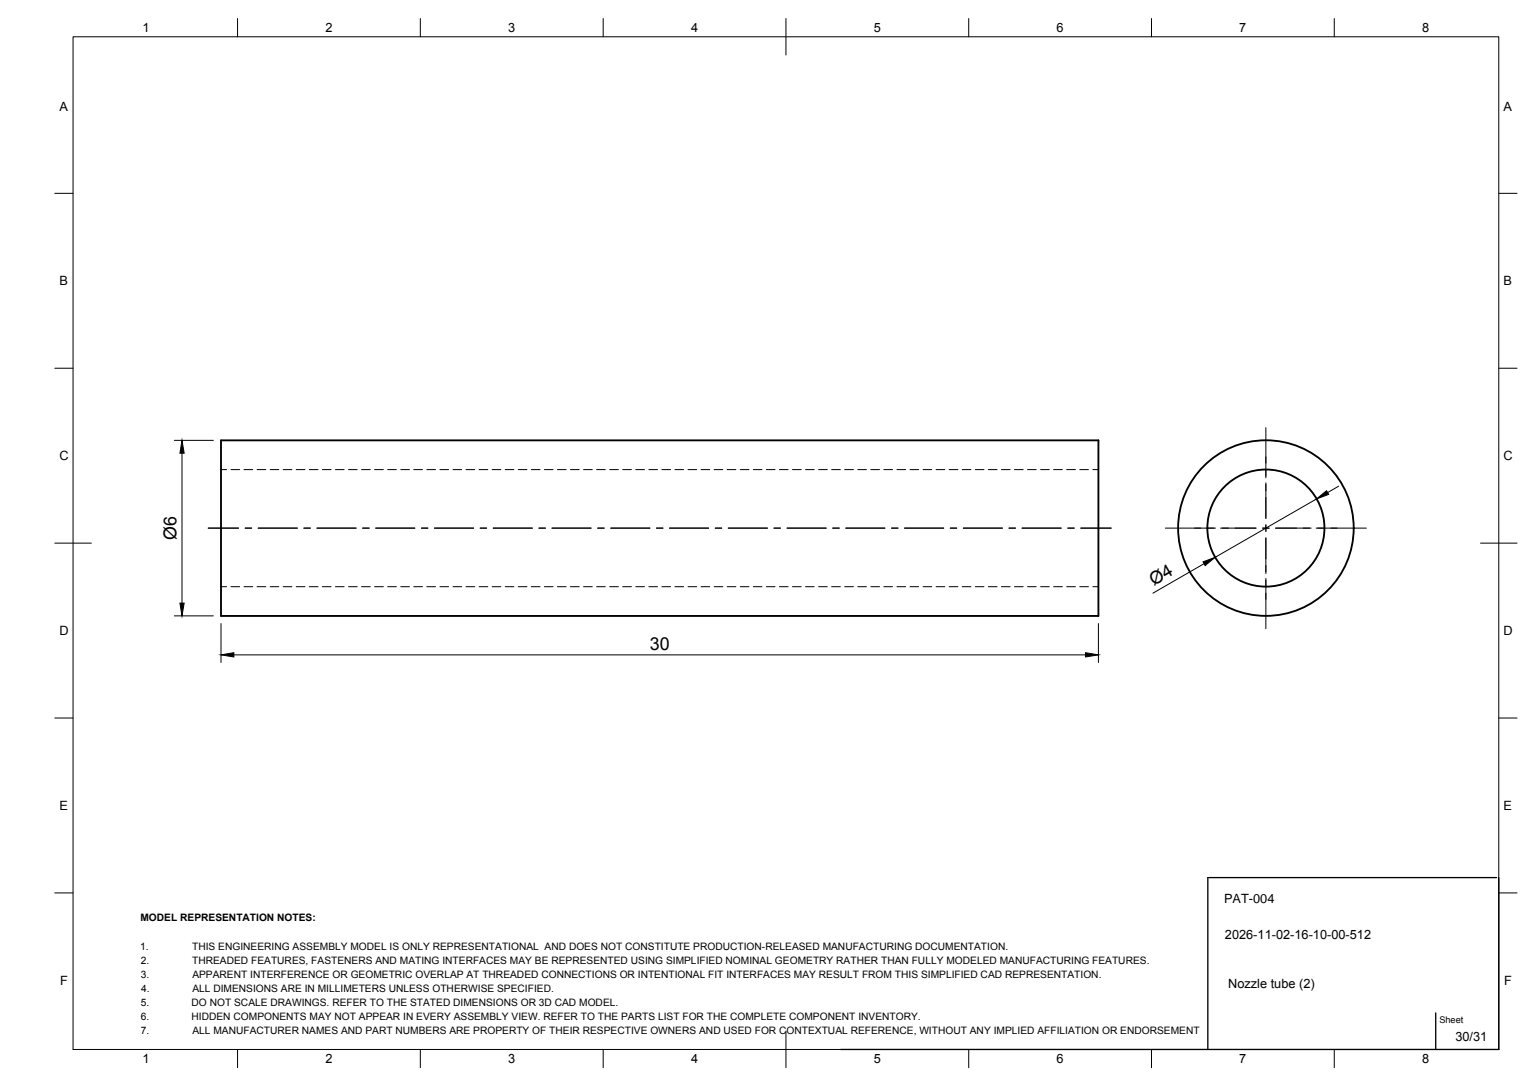
ISO-10303-21;
HEADER;
/* Generated by software containing ST-Developer
 * from STEP Tools, Inc. (www.steptools.com) 
 */

FILE_DESCRIPTION(
/* description */ ('Air blow-off nozzle station'),
/* implementation_level */ '2;1');

FILE_NAME(
/* name */ 'Nozzle tube (2).step',
/* time_stamp */ '2026-10-27T10:53:54-07:00',
/* author */ (''),
/* organization */ (''),
/* preprocessor_version */ 'ST-DEVELOPER v20.2',
/* originating_system */ 'Autodesk Translation Framework v15.17.0.0',
/* authorisation */ '');

FILE_SCHEMA (('AUTOMOTIVE_DESIGN { 1 0 10303 214 3 1 1 }'));
ENDSEC;

DATA;
#10=MECHANICAL_DESIGN_GEOMETRIC_PRESENTATION_REPRESENTATION('',(#258),#7897);
#208=SHAPE_REPRESENTATION_RELATIONSHIP('SRR','None',#8025,#233);
#233=ADVANCED_BREP_SHAPE_REPRESENTATION('',(#281),#7892);
#258=STYLED_ITEM('',(#8206),#281);
#281=MANIFOLD_SOLID_BREP('Body1',#4309);
#357=FACE_BOUND('',#1094,.T.);
#358=FACE_BOUND('',#1096,.T.);
#520=PLANE('',#4997);
#521=PLANE('',#4998);
#763=FACE_OUTER_BOUND('',#1091,.T.);
#764=FACE_OUTER_BOUND('',#1092,.T.);
#765=FACE_OUTER_BOUND('',#1093,.T.);
#766=FACE_OUTER_BOUND('',#1095,.T.);
#1091=EDGE_LOOP('',(#3845,#3846,#3847,#3848));
#1092=EDGE_LOOP('',(#3849,#3850,#3851,#3852));
#1093=EDGE_LOOP('',(#3853));
#1094=EDGE_LOOP('',(#3854));
#1095=EDGE_LOOP('',(#3855));
#1096=EDGE_LOOP('',(#3856));
#1461=LINE('',#7688,#1815);
#1462=LINE('',#7694,#1816);
#1815=VECTOR('',#6203,0.2);
#1816=VECTOR('',#6210,0.3);
#1981=CIRCLE('',#4992,0.2);
#1982=CIRCLE('',#4993,0.2);
#1983=CIRCLE('',#4995,0.3);
#1984=CIRCLE('',#4996,0.3);
#2328=VERTEX_POINT('',#7685);
#2329=VERTEX_POINT('',#7687);
#2330=VERTEX_POINT('',#7691);
#2331=VERTEX_POINT('',#7693);
#2840=EDGE_CURVE('',#2328,#2328,#1981,.T.);
#2841=EDGE_CURVE('',#2328,#2329,#1461,.T.);
#2842=EDGE_CURVE('',#2329,#2329,#1982,.T.);
#2843=EDGE_CURVE('',#2330,#2330,#1983,.T.);
#2844=EDGE_CURVE('',#2330,#2331,#1462,.T.);
#2845=EDGE_CURVE('',#2331,#2331,#1984,.T.);
#3845=ORIENTED_EDGE('',*,*,#2840,.F.);
#3846=ORIENTED_EDGE('',*,*,#2841,.T.);
#3847=ORIENTED_EDGE('',*,*,#2842,.T.);
#3848=ORIENTED_EDGE('',*,*,#2841,.F.);
#3849=ORIENTED_EDGE('',*,*,#2843,.F.);
#3850=ORIENTED_EDGE('',*,*,#2844,.T.);
#3851=ORIENTED_EDGE('',*,*,#2845,.T.);
#3852=ORIENTED_EDGE('',*,*,#2844,.F.);
#3853=ORIENTED_EDGE('',*,*,#2843,.T.);
#3854=ORIENTED_EDGE('',*,*,#2840,.T.);
#3855=ORIENTED_EDGE('',*,*,#2845,.F.);
#3856=ORIENTED_EDGE('',*,*,#2842,.F.);
#4017=CYLINDRICAL_SURFACE('',#4991,0.2);
#4018=CYLINDRICAL_SURFACE('',#4994,0.3);
#4253=ADVANCED_FACE('',(#763),#4017,.F.);
#4254=ADVANCED_FACE('',(#764),#4018,.T.);
#4255=ADVANCED_FACE('',(#765,#357),#520,.T.);
#4256=ADVANCED_FACE('',(#766,#358),#521,.F.);
#4309=CLOSED_SHELL('',(#4253,#4254,#4255,#4256));
#4990=AXIS2_PLACEMENT_3D('',#7683,#6197,#6198);
#4991=AXIS2_PLACEMENT_3D('',#7684,#6199,#6200);
#4992=AXIS2_PLACEMENT_3D('',#7686,#6201,#6202);
#4993=AXIS2_PLACEMENT_3D('',#7689,#6204,#6205);
#4994=AXIS2_PLACEMENT_3D('',#7690,#6206,#6207);
#4995=AXIS2_PLACEMENT_3D('',#7692,#6208,#6209);
#4996=AXIS2_PLACEMENT_3D('',#7695,#6211,#6212);
#4997=AXIS2_PLACEMENT_3D('',#7696,#6213,#6214);
#4998=AXIS2_PLACEMENT_3D('',#7697,#6215,#6216);
#6197=DIRECTION('axis',(0.,0.,1.));
#6198=DIRECTION('refdir',(1.,0.,0.));
#6199=DIRECTION('center_axis',(0.,1.,0.));
#6200=DIRECTION('ref_axis',(1.,0.,0.));
#6201=DIRECTION('center_axis',(0.,-1.,0.));
#6202=DIRECTION('ref_axis',(1.,0.,0.));
#6203=DIRECTION('',(0.,-1.,0.));
#6204=DIRECTION('center_axis',(0.,-1.,0.));
#6205=DIRECTION('ref_axis',(1.,0.,0.));
#6206=DIRECTION('center_axis',(0.,1.,0.));
#6207=DIRECTION('ref_axis',(1.,0.,0.));
#6208=DIRECTION('center_axis',(0.,1.,0.));
#6209=DIRECTION('ref_axis',(1.,0.,0.));
#6210=DIRECTION('',(0.,-1.,0.));
#6211=DIRECTION('center_axis',(0.,1.,0.));
#6212=DIRECTION('ref_axis',(1.,0.,0.));
#6213=DIRECTION('center_axis',(0.,1.,0.));
#6214=DIRECTION('ref_axis',(1.,0.,0.));
#6215=DIRECTION('center_axis',(0.,1.,0.));
#6216=DIRECTION('ref_axis',(1.,0.,0.));
#7683=CARTESIAN_POINT('',(0.,0.,0.));
#7684=CARTESIAN_POINT('Origin',(3.,-7.2,23.));
#7685=CARTESIAN_POINT('',(2.8,-4.2,23.));
#7686=CARTESIAN_POINT('Origin',(3.,-4.2,23.));
#7687=CARTESIAN_POINT('',(2.8,-7.2,23.));
#7688=CARTESIAN_POINT('',(2.8,-7.2,23.));
#7689=CARTESIAN_POINT('Origin',(3.,-7.2,23.));
#7690=CARTESIAN_POINT('Origin',(3.,-7.2,23.));
#7691=CARTESIAN_POINT('',(2.7,-4.2,23.));
#7692=CARTESIAN_POINT('Origin',(3.,-4.2,23.));
#7693=CARTESIAN_POINT('',(2.7,-7.2,23.));
#7694=CARTESIAN_POINT('',(2.7,-7.2,23.));
#7695=CARTESIAN_POINT('Origin',(3.,-7.2,23.));
#7696=CARTESIAN_POINT('Origin',(3.,-4.2,23.));
#7697=CARTESIAN_POINT('Origin',(3.,-7.2,23.));
#7860=UNCERTAINTY_MEASURE_WITH_UNIT(LENGTH_MEASURE(0.001),#7898,
'DISTANCE_ACCURACY_VALUE',
'Maximum model space distance between geometric entities at asserted c
onnectivities');
#7865=UNCERTAINTY_MEASURE_WITH_UNIT(LENGTH_MEASURE(0.001),#7898,
'DISTANCE_ACCURACY_VALUE',
'Maximum model space distance between geometric entities at asserted c
onnectivities');
#7892=(
GEOMETRIC_REPRESENTATION_CONTEXT(3)
GLOBAL_UNCERTAINTY_ASSIGNED_CONTEXT((#7860))
GLOBAL_UNIT_ASSIGNED_CONTEXT((#7898,#7900,#7901))
REPRESENTATION_CONTEXT('','3D')
);
#7897=(
GEOMETRIC_REPRESENTATION_CONTEXT(3)
GLOBAL_UNCERTAINTY_ASSIGNED_CONTEXT((#7865))
GLOBAL_UNIT_ASSIGNED_CONTEXT((#7898,#7900,#7901))
REPRESENTATION_CONTEXT('','3D')
);
#7898=(
LENGTH_UNIT()
NAMED_UNIT(*)
SI_UNIT(.CENTI.,.METRE.)
);
#7900=(
NAMED_UNIT(*)
PLANE_ANGLE_UNIT()
SI_UNIT($,.RADIAN.)
);
#7901=(
NAMED_UNIT(*)
SI_UNIT($,.STERADIAN.)
SOLID_ANGLE_UNIT()
);
#7928=SHAPE_DEFINITION_REPRESENTATION(#7976,#8025);
#7976=PRODUCT_DEFINITION_SHAPE('',$,#8057);
#8025=SHAPE_REPRESENTATION('',(#4990),#7892);
#8030=PRODUCT_DEFINITION_CONTEXT('part definition',#8125,'design');
#8057=PRODUCT_DEFINITION('Nozzle tube (2)','Nozzle tube (2)',#8088,#8030);
#8088=PRODUCT_DEFINITION_FORMATION('',$,#8153);
#8125=APPLICATION_CONTEXT(
'Core Data for Automotive Mechanical Design Process');
#8126=PRODUCT_CONTEXT('part definition',#8125,'mechanical');
#8153=PRODUCT('Nozzle tube (2)','Nozzle tube (2)','Nozzle tube (2)',(#8126));
#8200=COLOUR_RGB('Light Blue',0.38,0.62,0.78);
#8201=FILL_AREA_STYLE_COLOUR('',#8200);
#8202=FILL_AREA_STYLE('',(#8201));
#8203=SURFACE_STYLE_FILL_AREA(#8202);
#8204=SURFACE_SIDE_STYLE('',(#8203));
#8205=SURFACE_STYLE_USAGE(.BOTH.,#8204);
#8206=PRESENTATION_STYLE_ASSIGNMENT((#8205));
ENDSEC;
END-ISO-10303-21;
